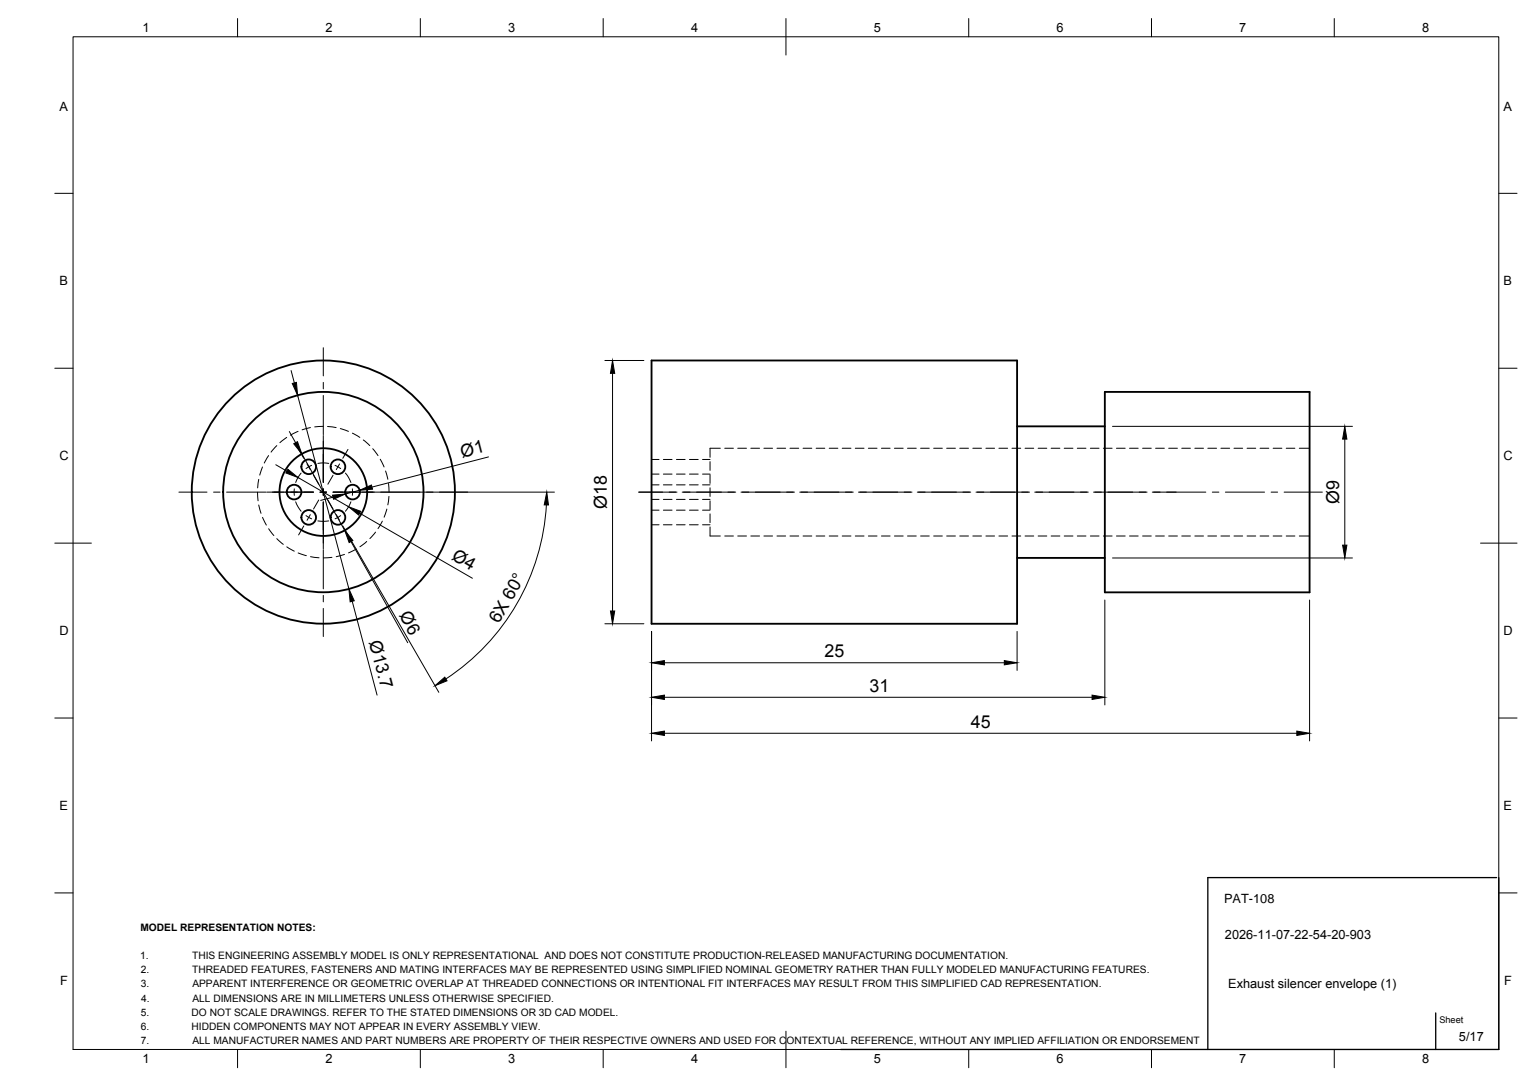
ISO-10303-21;
HEADER;
/* Generated by software containing ST-Developer
 * from STEP Tools, Inc. (www.steptools.com) 
 */

FILE_DESCRIPTION(
/* description */ ('Sub-base valve envelopes and connections'),
/* implementation_level */ '2;1');

FILE_NAME(
/* name */ 'Exhaust silencer envelope (1).step',
/* time_stamp */ '2026-10-29T15:55:44-07:00',
/* author */ (''),
/* organization */ (''),
/* preprocessor_version */ 'ST-DEVELOPER v20.2',
/* originating_system */ 'Autodesk Translation Framework v15.17.0.0',
/* authorisation */ '');

FILE_SCHEMA (('AUTOMOTIVE_DESIGN { 1 0 10303 214 3 1 1 }'));
ENDSEC;

DATA;
#10=MECHANICAL_DESIGN_GEOMETRIC_PRESENTATION_REPRESENTATION('',(#121),#6113);
#97=SHAPE_REPRESENTATION_RELATIONSHIP('SRR','None',#6170,#109);
#109=ADVANCED_BREP_SHAPE_REPRESENTATION('',(#133),#6101);
#121=STYLED_ITEM('',(#6329),#133);
#133=MANIFOLD_SOLID_BREP('Body1',#3360);
#191=FACE_BOUND('',#703,.T.);
#192=FACE_BOUND('',#704,.T.);
#193=FACE_BOUND('',#705,.T.);
#194=FACE_BOUND('',#706,.T.);
#195=FACE_BOUND('',#707,.T.);
#196=FACE_BOUND('',#708,.T.);
#197=FACE_BOUND('',#710,.T.);
#198=FACE_BOUND('',#713,.T.);
#199=FACE_BOUND('',#714,.T.);
#200=FACE_BOUND('',#715,.T.);
#201=FACE_BOUND('',#716,.T.);
#202=FACE_BOUND('',#717,.T.);
#203=FACE_BOUND('',#718,.T.);
#204=FACE_BOUND('',#723,.T.);
#205=FACE_BOUND('',#725,.T.);
#302=PLANE('',#3656);
#303=PLANE('',#3658);
#304=PLANE('',#3663);
#305=PLANE('',#3671);
#306=PLANE('',#3672);
#448=FACE_OUTER_BOUND('',#696,.T.);
#449=FACE_OUTER_BOUND('',#697,.T.);
#450=FACE_OUTER_BOUND('',#698,.T.);
#451=FACE_OUTER_BOUND('',#699,.T.);
#452=FACE_OUTER_BOUND('',#700,.T.);
#453=FACE_OUTER_BOUND('',#701,.T.);
#454=FACE_OUTER_BOUND('',#702,.T.);
#455=FACE_OUTER_BOUND('',#709,.T.);
#456=FACE_OUTER_BOUND('',#711,.T.);
#457=FACE_OUTER_BOUND('',#712,.T.);
#458=FACE_OUTER_BOUND('',#719,.T.);
#459=FACE_OUTER_BOUND('',#720,.T.);
#460=FACE_OUTER_BOUND('',#721,.T.);
#461=FACE_OUTER_BOUND('',#722,.T.);
#462=FACE_OUTER_BOUND('',#724,.T.);
#696=EDGE_LOOP('',(#2517,#2518,#2519,#2520));
#697=EDGE_LOOP('',(#2521,#2522,#2523,#2524));
#698=EDGE_LOOP('',(#2525,#2526,#2527,#2528));
#699=EDGE_LOOP('',(#2529,#2530,#2531,#2532));
#700=EDGE_LOOP('',(#2533,#2534,#2535,#2536));
#701=EDGE_LOOP('',(#2537,#2538,#2539,#2540));
#702=EDGE_LOOP('',(#2541));
#703=EDGE_LOOP('',(#2542));
#704=EDGE_LOOP('',(#2543));
#705=EDGE_LOOP('',(#2544));
#706=EDGE_LOOP('',(#2545));
#707=EDGE_LOOP('',(#2546));
#708=EDGE_LOOP('',(#2547));
#709=EDGE_LOOP('',(#2548));
#710=EDGE_LOOP('',(#2549));
#711=EDGE_LOOP('',(#2550,#2551,#2552,#2553));
#712=EDGE_LOOP('',(#2554));
#713=EDGE_LOOP('',(#2555));
#714=EDGE_LOOP('',(#2556));
#715=EDGE_LOOP('',(#2557));
#716=EDGE_LOOP('',(#2558));
#717=EDGE_LOOP('',(#2559));
#718=EDGE_LOOP('',(#2560));
#719=EDGE_LOOP('',(#2561,#2562,#2563,#2564));
#720=EDGE_LOOP('',(#2565,#2566,#2567,#2568));
#721=EDGE_LOOP('',(#2569,#2570,#2571,#2572));
#722=EDGE_LOOP('',(#2573));
#723=EDGE_LOOP('',(#2574));
#724=EDGE_LOOP('',(#2575));
#725=EDGE_LOOP('',(#2576));
#956=LINE('',#5456,#1190);
#957=LINE('',#5462,#1191);
#958=LINE('',#5468,#1192);
#959=LINE('',#5474,#1193);
#960=LINE('',#5480,#1194);
#961=LINE('',#5486,#1195);
#962=LINE('',#5499,#1196);
#963=LINE('',#5503,#1197);
#964=LINE('',#5507,#1198);
#965=LINE('',#5513,#1199);
#1190=VECTOR('',#4232,0.05);
#1191=VECTOR('',#4239,0.05);
#1192=VECTOR('',#4246,0.05);
#1193=VECTOR('',#4253,0.05);
#1194=VECTOR('',#4260,0.05);
#1195=VECTOR('',#4267,0.05);
#1196=VECTOR('',#4284,0.9);
#1197=VECTOR('',#4289,0.45);
#1198=VECTOR('',#4294,0.3);
#1199=VECTOR('',#4301,0.685);
#1437=CIRCLE('',#3639,0.05);
#1438=CIRCLE('',#3640,0.05);
#1439=CIRCLE('',#3642,0.05);
#1440=CIRCLE('',#3643,0.05);
#1441=CIRCLE('',#3645,0.05);
#1442=CIRCLE('',#3646,0.05);
#1443=CIRCLE('',#3648,0.05);
#1444=CIRCLE('',#3649,0.05);
#1445=CIRCLE('',#3651,0.05);
#1446=CIRCLE('',#3652,0.05);
#1447=CIRCLE('',#3654,0.05);
#1448=CIRCLE('',#3655,0.05);
#1449=CIRCLE('',#3657,0.3);
#1450=CIRCLE('',#3659,0.9);
#1451=CIRCLE('',#3660,0.45);
#1452=CIRCLE('',#3662,0.9);
#1453=CIRCLE('',#3665,0.45);
#1454=CIRCLE('',#3667,0.3);
#1455=CIRCLE('',#3669,0.685);
#1456=CIRCLE('',#3670,0.685);
#1631=VERTEX_POINT('',#5453);
#1632=VERTEX_POINT('',#5455);
#1633=VERTEX_POINT('',#5459);
#1634=VERTEX_POINT('',#5461);
#1635=VERTEX_POINT('',#5465);
#1636=VERTEX_POINT('',#5467);
#1637=VERTEX_POINT('',#5471);
#1638=VERTEX_POINT('',#5473);
#1639=VERTEX_POINT('',#5477);
#1640=VERTEX_POINT('',#5479);
#1641=VERTEX_POINT('',#5483);
#1642=VERTEX_POINT('',#5485);
#1643=VERTEX_POINT('',#5489);
#1644=VERTEX_POINT('',#5492);
#1645=VERTEX_POINT('',#5494);
#1646=VERTEX_POINT('',#5497);
#1647=VERTEX_POINT('',#5502);
#1648=VERTEX_POINT('',#5506);
#1649=VERTEX_POINT('',#5510);
#1650=VERTEX_POINT('',#5512);
#1956=EDGE_CURVE('',#1631,#1631,#1437,.T.);
#1957=EDGE_CURVE('',#1631,#1632,#956,.T.);
#1958=EDGE_CURVE('',#1632,#1632,#1438,.T.);
#1959=EDGE_CURVE('',#1633,#1633,#1439,.T.);
#1960=EDGE_CURVE('',#1633,#1634,#957,.T.);
#1961=EDGE_CURVE('',#1634,#1634,#1440,.T.);
#1962=EDGE_CURVE('',#1635,#1635,#1441,.T.);
#1963=EDGE_CURVE('',#1635,#1636,#958,.T.);
#1964=EDGE_CURVE('',#1636,#1636,#1442,.T.);
#1965=EDGE_CURVE('',#1637,#1637,#1443,.T.);
#1966=EDGE_CURVE('',#1637,#1638,#959,.T.);
#1967=EDGE_CURVE('',#1638,#1638,#1444,.T.);
#1968=EDGE_CURVE('',#1639,#1639,#1445,.T.);
#1969=EDGE_CURVE('',#1639,#1640,#960,.T.);
#1970=EDGE_CURVE('',#1640,#1640,#1446,.T.);
#1971=EDGE_CURVE('',#1641,#1641,#1447,.T.);
#1972=EDGE_CURVE('',#1641,#1642,#961,.T.);
#1973=EDGE_CURVE('',#1642,#1642,#1448,.T.);
#1974=EDGE_CURVE('',#1643,#1643,#1449,.T.);
#1975=EDGE_CURVE('',#1644,#1644,#1450,.T.);
#1976=EDGE_CURVE('',#1645,#1645,#1451,.T.);
#1977=EDGE_CURVE('',#1646,#1646,#1452,.T.);
#1978=EDGE_CURVE('',#1646,#1644,#962,.T.);
#1979=EDGE_CURVE('',#1645,#1647,#963,.T.);
#1980=EDGE_CURVE('',#1647,#1647,#1453,.T.);
#1981=EDGE_CURVE('',#1643,#1648,#964,.T.);
#1982=EDGE_CURVE('',#1648,#1648,#1454,.T.);
#1983=EDGE_CURVE('',#1649,#1649,#1455,.T.);
#1984=EDGE_CURVE('',#1649,#1650,#965,.T.);
#1985=EDGE_CURVE('',#1650,#1650,#1456,.T.);
#2517=ORIENTED_EDGE('',*,*,#1956,.F.);
#2518=ORIENTED_EDGE('',*,*,#1957,.T.);
#2519=ORIENTED_EDGE('',*,*,#1958,.F.);
#2520=ORIENTED_EDGE('',*,*,#1957,.F.);
#2521=ORIENTED_EDGE('',*,*,#1959,.F.);
#2522=ORIENTED_EDGE('',*,*,#1960,.T.);
#2523=ORIENTED_EDGE('',*,*,#1961,.F.);
#2524=ORIENTED_EDGE('',*,*,#1960,.F.);
#2525=ORIENTED_EDGE('',*,*,#1962,.F.);
#2526=ORIENTED_EDGE('',*,*,#1963,.T.);
#2527=ORIENTED_EDGE('',*,*,#1964,.F.);
#2528=ORIENTED_EDGE('',*,*,#1963,.F.);
#2529=ORIENTED_EDGE('',*,*,#1965,.F.);
#2530=ORIENTED_EDGE('',*,*,#1966,.T.);
#2531=ORIENTED_EDGE('',*,*,#1967,.F.);
#2532=ORIENTED_EDGE('',*,*,#1966,.F.);
#2533=ORIENTED_EDGE('',*,*,#1968,.F.);
#2534=ORIENTED_EDGE('',*,*,#1969,.T.);
#2535=ORIENTED_EDGE('',*,*,#1970,.F.);
#2536=ORIENTED_EDGE('',*,*,#1969,.F.);
#2537=ORIENTED_EDGE('',*,*,#1971,.F.);
#2538=ORIENTED_EDGE('',*,*,#1972,.T.);
#2539=ORIENTED_EDGE('',*,*,#1973,.F.);
#2540=ORIENTED_EDGE('',*,*,#1972,.F.);
#2541=ORIENTED_EDGE('',*,*,#1974,.F.);
#2542=ORIENTED_EDGE('',*,*,#1971,.T.);
#2543=ORIENTED_EDGE('',*,*,#1968,.T.);
#2544=ORIENTED_EDGE('',*,*,#1965,.T.);
#2545=ORIENTED_EDGE('',*,*,#1962,.T.);
#2546=ORIENTED_EDGE('',*,*,#1959,.T.);
#2547=ORIENTED_EDGE('',*,*,#1956,.T.);
#2548=ORIENTED_EDGE('',*,*,#1975,.F.);
#2549=ORIENTED_EDGE('',*,*,#1976,.F.);
#2550=ORIENTED_EDGE('',*,*,#1977,.F.);
#2551=ORIENTED_EDGE('',*,*,#1978,.T.);
#2552=ORIENTED_EDGE('',*,*,#1975,.T.);
#2553=ORIENTED_EDGE('',*,*,#1978,.F.);
#2554=ORIENTED_EDGE('',*,*,#1977,.T.);
#2555=ORIENTED_EDGE('',*,*,#1973,.T.);
#2556=ORIENTED_EDGE('',*,*,#1970,.T.);
#2557=ORIENTED_EDGE('',*,*,#1967,.T.);
#2558=ORIENTED_EDGE('',*,*,#1964,.T.);
#2559=ORIENTED_EDGE('',*,*,#1961,.T.);
#2560=ORIENTED_EDGE('',*,*,#1958,.T.);
#2561=ORIENTED_EDGE('',*,*,#1976,.T.);
#2562=ORIENTED_EDGE('',*,*,#1979,.T.);
#2563=ORIENTED_EDGE('',*,*,#1980,.F.);
#2564=ORIENTED_EDGE('',*,*,#1979,.F.);
#2565=ORIENTED_EDGE('',*,*,#1974,.T.);
#2566=ORIENTED_EDGE('',*,*,#1981,.T.);
#2567=ORIENTED_EDGE('',*,*,#1982,.T.);
#2568=ORIENTED_EDGE('',*,*,#1981,.F.);
#2569=ORIENTED_EDGE('',*,*,#1983,.F.);
#2570=ORIENTED_EDGE('',*,*,#1984,.T.);
#2571=ORIENTED_EDGE('',*,*,#1985,.T.);
#2572=ORIENTED_EDGE('',*,*,#1984,.F.);
#2573=ORIENTED_EDGE('',*,*,#1983,.T.);
#2574=ORIENTED_EDGE('',*,*,#1980,.T.);
#2575=ORIENTED_EDGE('',*,*,#1985,.F.);
#2576=ORIENTED_EDGE('',*,*,#1982,.F.);
#3112=CYLINDRICAL_SURFACE('',#3638,0.05);
#3113=CYLINDRICAL_SURFACE('',#3641,0.05);
#3114=CYLINDRICAL_SURFACE('',#3644,0.05);
#3115=CYLINDRICAL_SURFACE('',#3647,0.05);
#3116=CYLINDRICAL_SURFACE('',#3650,0.05);
#3117=CYLINDRICAL_SURFACE('',#3653,0.05);
#3118=CYLINDRICAL_SURFACE('',#3661,0.9);
#3119=CYLINDRICAL_SURFACE('',#3664,0.45);
#3120=CYLINDRICAL_SURFACE('',#3666,0.3);
#3121=CYLINDRICAL_SURFACE('',#3668,0.685);
#3221=ADVANCED_FACE('',(#448),#3112,.F.);
#3222=ADVANCED_FACE('',(#449),#3113,.F.);
#3223=ADVANCED_FACE('',(#450),#3114,.F.);
#3224=ADVANCED_FACE('',(#451),#3115,.F.);
#3225=ADVANCED_FACE('',(#452),#3116,.F.);
#3226=ADVANCED_FACE('',(#453),#3117,.F.);
#3227=ADVANCED_FACE('',(#454,#191,#192,#193,#194,#195,#196),#302,.F.);
#3228=ADVANCED_FACE('',(#455,#197),#303,.F.);
#3229=ADVANCED_FACE('',(#456),#3118,.T.);
#3230=ADVANCED_FACE('',(#457,#198,#199,#200,#201,#202,#203),#304,.T.);
#3231=ADVANCED_FACE('',(#458),#3119,.T.);
#3232=ADVANCED_FACE('',(#459),#3120,.F.);
#3233=ADVANCED_FACE('',(#460),#3121,.T.);
#3234=ADVANCED_FACE('',(#461,#204),#305,.T.);
#3235=ADVANCED_FACE('',(#462,#205),#306,.F.);
#3360=CLOSED_SHELL('',(#3221,#3222,#3223,#3224,#3225,#3226,#3227,#3228,
#3229,#3230,#3231,#3232,#3233,#3234,#3235));
#3637=AXIS2_PLACEMENT_3D('',#5451,#4226,#4227);
#3638=AXIS2_PLACEMENT_3D('',#5452,#4228,#4229);
#3639=AXIS2_PLACEMENT_3D('',#5454,#4230,#4231);
#3640=AXIS2_PLACEMENT_3D('',#5457,#4233,#4234);
#3641=AXIS2_PLACEMENT_3D('',#5458,#4235,#4236);
#3642=AXIS2_PLACEMENT_3D('',#5460,#4237,#4238);
#3643=AXIS2_PLACEMENT_3D('',#5463,#4240,#4241);
#3644=AXIS2_PLACEMENT_3D('',#5464,#4242,#4243);
#3645=AXIS2_PLACEMENT_3D('',#5466,#4244,#4245);
#3646=AXIS2_PLACEMENT_3D('',#5469,#4247,#4248);
#3647=AXIS2_PLACEMENT_3D('',#5470,#4249,#4250);
#3648=AXIS2_PLACEMENT_3D('',#5472,#4251,#4252);
#3649=AXIS2_PLACEMENT_3D('',#5475,#4254,#4255);
#3650=AXIS2_PLACEMENT_3D('',#5476,#4256,#4257);
#3651=AXIS2_PLACEMENT_3D('',#5478,#4258,#4259);
#3652=AXIS2_PLACEMENT_3D('',#5481,#4261,#4262);
#3653=AXIS2_PLACEMENT_3D('',#5482,#4263,#4264);
#3654=AXIS2_PLACEMENT_3D('',#5484,#4265,#4266);
#3655=AXIS2_PLACEMENT_3D('',#5487,#4268,#4269);
#3656=AXIS2_PLACEMENT_3D('',#5488,#4270,#4271);
#3657=AXIS2_PLACEMENT_3D('',#5490,#4272,#4273);
#3658=AXIS2_PLACEMENT_3D('',#5491,#4274,#4275);
#3659=AXIS2_PLACEMENT_3D('',#5493,#4276,#4277);
#3660=AXIS2_PLACEMENT_3D('',#5495,#4278,#4279);
#3661=AXIS2_PLACEMENT_3D('',#5496,#4280,#4281);
#3662=AXIS2_PLACEMENT_3D('',#5498,#4282,#4283);
#3663=AXIS2_PLACEMENT_3D('',#5500,#4285,#4286);
#3664=AXIS2_PLACEMENT_3D('',#5501,#4287,#4288);
#3665=AXIS2_PLACEMENT_3D('',#5504,#4290,#4291);
#3666=AXIS2_PLACEMENT_3D('',#5505,#4292,#4293);
#3667=AXIS2_PLACEMENT_3D('',#5508,#4295,#4296);
#3668=AXIS2_PLACEMENT_3D('',#5509,#4297,#4298);
#3669=AXIS2_PLACEMENT_3D('',#5511,#4299,#4300);
#3670=AXIS2_PLACEMENT_3D('',#5514,#4302,#4303);
#3671=AXIS2_PLACEMENT_3D('',#5515,#4304,#4305);
#3672=AXIS2_PLACEMENT_3D('',#5516,#4306,#4307);
#4226=DIRECTION('axis',(0.,0.,1.));
#4227=DIRECTION('refdir',(1.,0.,0.));
#4228=DIRECTION('center_axis',(1.,0.,0.));
#4229=DIRECTION('ref_axis',(0.,0.,-1.));
#4230=DIRECTION('center_axis',(1.,0.,0.));
#4231=DIRECTION('ref_axis',(0.,0.,-1.));
#4232=DIRECTION('',(1.,0.,0.));
#4233=DIRECTION('center_axis',(-1.,0.,0.));
#4234=DIRECTION('ref_axis',(0.,0.,-1.));
#4235=DIRECTION('center_axis',(1.,0.,0.));
#4236=DIRECTION('ref_axis',(0.,0.,-1.));
#4237=DIRECTION('center_axis',(1.,0.,0.));
#4238=DIRECTION('ref_axis',(0.,0.,-1.));
#4239=DIRECTION('',(1.,0.,0.));
#4240=DIRECTION('center_axis',(-1.,0.,0.));
#4241=DIRECTION('ref_axis',(0.,0.,-1.));
#4242=DIRECTION('center_axis',(1.,0.,0.));
#4243=DIRECTION('ref_axis',(0.,0.,-1.));
#4244=DIRECTION('center_axis',(1.,0.,0.));
#4245=DIRECTION('ref_axis',(0.,0.,-1.));
#4246=DIRECTION('',(1.,0.,0.));
#4247=DIRECTION('center_axis',(-1.,0.,0.));
#4248=DIRECTION('ref_axis',(0.,0.,-1.));
#4249=DIRECTION('center_axis',(1.,0.,0.));
#4250=DIRECTION('ref_axis',(0.,0.,-1.));
#4251=DIRECTION('center_axis',(1.,0.,0.));
#4252=DIRECTION('ref_axis',(0.,0.,-1.));
#4253=DIRECTION('',(1.,0.,0.));
#4254=DIRECTION('center_axis',(-1.,0.,0.));
#4255=DIRECTION('ref_axis',(0.,0.,-1.));
#4256=DIRECTION('center_axis',(1.,0.,0.));
#4257=DIRECTION('ref_axis',(0.,0.,-1.));
#4258=DIRECTION('center_axis',(1.,0.,0.));
#4259=DIRECTION('ref_axis',(0.,0.,-1.));
#4260=DIRECTION('',(1.,0.,0.));
#4261=DIRECTION('center_axis',(-1.,0.,0.));
#4262=DIRECTION('ref_axis',(0.,0.,-1.));
#4263=DIRECTION('center_axis',(1.,0.,0.));
#4264=DIRECTION('ref_axis',(0.,0.,-1.));
#4265=DIRECTION('center_axis',(1.,0.,0.));
#4266=DIRECTION('ref_axis',(0.,0.,-1.));
#4267=DIRECTION('',(1.,0.,0.));
#4268=DIRECTION('center_axis',(-1.,0.,0.));
#4269=DIRECTION('ref_axis',(0.,0.,-1.));
#4270=DIRECTION('center_axis',(1.,0.,0.));
#4271=DIRECTION('ref_axis',(0.,0.,-1.));
#4272=DIRECTION('center_axis',(1.,0.,0.));
#4273=DIRECTION('ref_axis',(0.,0.,-1.));
#4274=DIRECTION('center_axis',(1.,0.,0.));
#4275=DIRECTION('ref_axis',(0.,0.,-1.));
#4276=DIRECTION('center_axis',(1.,0.,0.));
#4277=DIRECTION('ref_axis',(0.,0.,-1.));
#4278=DIRECTION('center_axis',(-1.,0.,0.));
#4279=DIRECTION('ref_axis',(0.,0.,-1.));
#4280=DIRECTION('center_axis',(1.,0.,0.));
#4281=DIRECTION('ref_axis',(0.,0.,-1.));
#4282=DIRECTION('center_axis',(1.,0.,0.));
#4283=DIRECTION('ref_axis',(0.,0.,-1.));
#4284=DIRECTION('',(-1.,0.,0.));
#4285=DIRECTION('center_axis',(1.,0.,0.));
#4286=DIRECTION('ref_axis',(0.,0.,-1.));
#4287=DIRECTION('center_axis',(1.,0.,0.));
#4288=DIRECTION('ref_axis',(0.,0.,-1.));
#4289=DIRECTION('',(-1.,0.,0.));
#4290=DIRECTION('center_axis',(-1.,0.,0.));
#4291=DIRECTION('ref_axis',(0.,0.,-1.));
#4292=DIRECTION('center_axis',(1.,0.,0.));
#4293=DIRECTION('ref_axis',(0.,0.,-1.));
#4294=DIRECTION('',(-1.,0.,0.));
#4295=DIRECTION('center_axis',(-1.,0.,0.));
#4296=DIRECTION('ref_axis',(0.,0.,-1.));
#4297=DIRECTION('center_axis',(1.,0.,0.));
#4298=DIRECTION('ref_axis',(0.,0.,-1.));
#4299=DIRECTION('center_axis',(1.,0.,0.));
#4300=DIRECTION('ref_axis',(0.,0.,-1.));
#4301=DIRECTION('',(-1.,0.,0.));
#4302=DIRECTION('center_axis',(1.,0.,0.));
#4303=DIRECTION('ref_axis',(0.,0.,-1.));
#4304=DIRECTION('center_axis',(1.,0.,0.));
#4305=DIRECTION('ref_axis',(0.,0.,-1.));
#4306=DIRECTION('center_axis',(1.,0.,0.));
#4307=DIRECTION('ref_axis',(0.,0.,-1.));
#5451=CARTESIAN_POINT('',(0.,0.,0.));
#5452=CARTESIAN_POINT('Origin',(10.6,1.4,0.826794919243112));
#5453=CARTESIAN_POINT('',(10.7,1.4,0.876794919243112));
#5454=CARTESIAN_POINT('Origin',(10.7,1.4,0.826794919243112));
#5455=CARTESIAN_POINT('',(11.1,1.4,0.876794919243112));
#5456=CARTESIAN_POINT('',(10.6,1.4,0.876794919243112));
#5457=CARTESIAN_POINT('Origin',(11.1,1.4,0.826794919243112));
#5458=CARTESIAN_POINT('Origin',(10.6,1.7,1.));
#5459=CARTESIAN_POINT('',(10.7,1.7,1.05));
#5460=CARTESIAN_POINT('Origin',(10.7,1.7,1.));
#5461=CARTESIAN_POINT('',(11.1,1.7,1.05));
#5462=CARTESIAN_POINT('',(10.6,1.7,1.05));
#5463=CARTESIAN_POINT('Origin',(11.1,1.7,1.));
#5464=CARTESIAN_POINT('Origin',(10.6,1.6,1.17320508075689));
#5465=CARTESIAN_POINT('',(10.7,1.6,1.22320508075689));
#5466=CARTESIAN_POINT('Origin',(10.7,1.6,1.17320508075689));
#5467=CARTESIAN_POINT('',(11.1,1.6,1.22320508075689));
#5468=CARTESIAN_POINT('',(10.6,1.6,1.22320508075689));
#5469=CARTESIAN_POINT('Origin',(11.1,1.6,1.17320508075689));
#5470=CARTESIAN_POINT('Origin',(10.6,1.4,1.17320508075689));
#5471=CARTESIAN_POINT('',(10.7,1.4,1.22320508075689));
#5472=CARTESIAN_POINT('Origin',(10.7,1.4,1.17320508075689));
#5473=CARTESIAN_POINT('',(11.1,1.4,1.22320508075689));
#5474=CARTESIAN_POINT('',(10.6,1.4,1.22320508075689));
#5475=CARTESIAN_POINT('Origin',(11.1,1.4,1.17320508075689));
#5476=CARTESIAN_POINT('Origin',(10.6,1.3,1.));
#5477=CARTESIAN_POINT('',(10.7,1.3,1.05));
#5478=CARTESIAN_POINT('Origin',(10.7,1.3,1.));
#5479=CARTESIAN_POINT('',(11.1,1.3,1.05));
#5480=CARTESIAN_POINT('',(10.6,1.3,1.05));
#5481=CARTESIAN_POINT('Origin',(11.1,1.3,1.));
#5482=CARTESIAN_POINT('Origin',(10.6,1.6,0.826794919243112));
#5483=CARTESIAN_POINT('',(10.7,1.6,0.876794919243112));
#5484=CARTESIAN_POINT('Origin',(10.7,1.6,0.826794919243112));
#5485=CARTESIAN_POINT('',(11.1,1.6,0.876794919243112));
#5486=CARTESIAN_POINT('',(10.6,1.6,0.876794919243112));
#5487=CARTESIAN_POINT('Origin',(11.1,1.6,0.826794919243112));
#5488=CARTESIAN_POINT('Origin',(10.7,1.5,1.));
#5489=CARTESIAN_POINT('',(10.7,1.5,1.3));
#5490=CARTESIAN_POINT('Origin',(10.7,1.5,1.));
#5491=CARTESIAN_POINT('Origin',(8.6,1.5,1.));
#5492=CARTESIAN_POINT('',(8.6,1.5,1.9));
#5493=CARTESIAN_POINT('Origin',(8.6,1.5,1.));
#5494=CARTESIAN_POINT('',(8.6,1.5,1.45));
#5495=CARTESIAN_POINT('Origin',(8.6,1.5,1.));
#5496=CARTESIAN_POINT('Origin',(8.6,1.5,1.));
#5497=CARTESIAN_POINT('',(11.1,1.5,1.9));
#5498=CARTESIAN_POINT('Origin',(11.1,1.5,1.));
#5499=CARTESIAN_POINT('',(8.6,1.5,1.9));
#5500=CARTESIAN_POINT('Origin',(11.1,1.5,1.));
#5501=CARTESIAN_POINT('Origin',(8.,1.5,1.));
#5502=CARTESIAN_POINT('',(8.,1.5,1.45));
#5503=CARTESIAN_POINT('',(8.,1.5,1.45));
#5504=CARTESIAN_POINT('Origin',(8.,1.5,1.));
#5505=CARTESIAN_POINT('Origin',(6.6,1.5,1.));
#5506=CARTESIAN_POINT('',(6.6,1.5,1.3));
#5507=CARTESIAN_POINT('',(6.6,1.5,1.3));
#5508=CARTESIAN_POINT('Origin',(6.6,1.5,1.));
#5509=CARTESIAN_POINT('Origin',(6.6,1.5,1.));
#5510=CARTESIAN_POINT('',(8.,1.5,1.685));
#5511=CARTESIAN_POINT('Origin',(8.,1.5,1.));
#5512=CARTESIAN_POINT('',(6.6,1.5,1.685));
#5513=CARTESIAN_POINT('',(6.6,1.5,1.685));
#5514=CARTESIAN_POINT('Origin',(6.6,1.5,1.));
#5515=CARTESIAN_POINT('Origin',(8.,1.5,1.));
#5516=CARTESIAN_POINT('Origin',(6.6,1.5,1.));
#6085=UNCERTAINTY_MEASURE_WITH_UNIT(LENGTH_MEASURE(0.001),#6114,
'DISTANCE_ACCURACY_VALUE',
'Maximum model space distance between geometric entities at asserted c
onnectivities');
#6097=UNCERTAINTY_MEASURE_WITH_UNIT(LENGTH_MEASURE(0.001),#6114,
'DISTANCE_ACCURACY_VALUE',
'Maximum model space distance between geometric entities at asserted c
onnectivities');
#6101=(
GEOMETRIC_REPRESENTATION_CONTEXT(3)
GLOBAL_UNCERTAINTY_ASSIGNED_CONTEXT((#6085))
GLOBAL_UNIT_ASSIGNED_CONTEXT((#6114,#6116,#6117))
REPRESENTATION_CONTEXT('','3D')
);
#6113=(
GEOMETRIC_REPRESENTATION_CONTEXT(3)
GLOBAL_UNCERTAINTY_ASSIGNED_CONTEXT((#6097))
GLOBAL_UNIT_ASSIGNED_CONTEXT((#6114,#6116,#6117))
REPRESENTATION_CONTEXT('','3D')
);
#6114=(
LENGTH_UNIT()
NAMED_UNIT(*)
SI_UNIT(.CENTI.,.METRE.)
);
#6116=(
NAMED_UNIT(*)
PLANE_ANGLE_UNIT()
SI_UNIT($,.RADIAN.)
);
#6117=(
NAMED_UNIT(*)
SI_UNIT($,.STERADIAN.)
SOLID_ANGLE_UNIT()
);
#6121=SHAPE_DEFINITION_REPRESENTATION(#6136,#6170);
#6136=PRODUCT_DEFINITION_SHAPE('',$,#6186);
#6170=SHAPE_REPRESENTATION('',(#3637),#6101);
#6182=PRODUCT_DEFINITION_CONTEXT('part definition',#6229,'design');
#6186=PRODUCT_DEFINITION('Exhaust silencer envelope (1)',
'Exhaust silencer envelope (1)',#6201,#6182);
#6201=PRODUCT_DEFINITION_FORMATION('',$,#6234);
#6229=APPLICATION_CONTEXT(
'Core Data for Automotive Mechanical Design Process');
#6230=PRODUCT_CONTEXT('part definition',#6229,'mechanical');
#6234=PRODUCT('Exhaust silencer envelope (1)',
'Exhaust silencer envelope (1)','Exhaust silencer envelope (1)',(#6230));
#6323=COLOUR_RGB('Off White',0.89,0.88,0.83);
#6324=FILL_AREA_STYLE_COLOUR('',#6323);
#6325=FILL_AREA_STYLE('',(#6324));
#6326=SURFACE_STYLE_FILL_AREA(#6325);
#6327=SURFACE_SIDE_STYLE('',(#6326));
#6328=SURFACE_STYLE_USAGE(.BOTH.,#6327);
#6329=PRESENTATION_STYLE_ASSIGNMENT((#6328));
ENDSEC;
END-ISO-10303-21;
